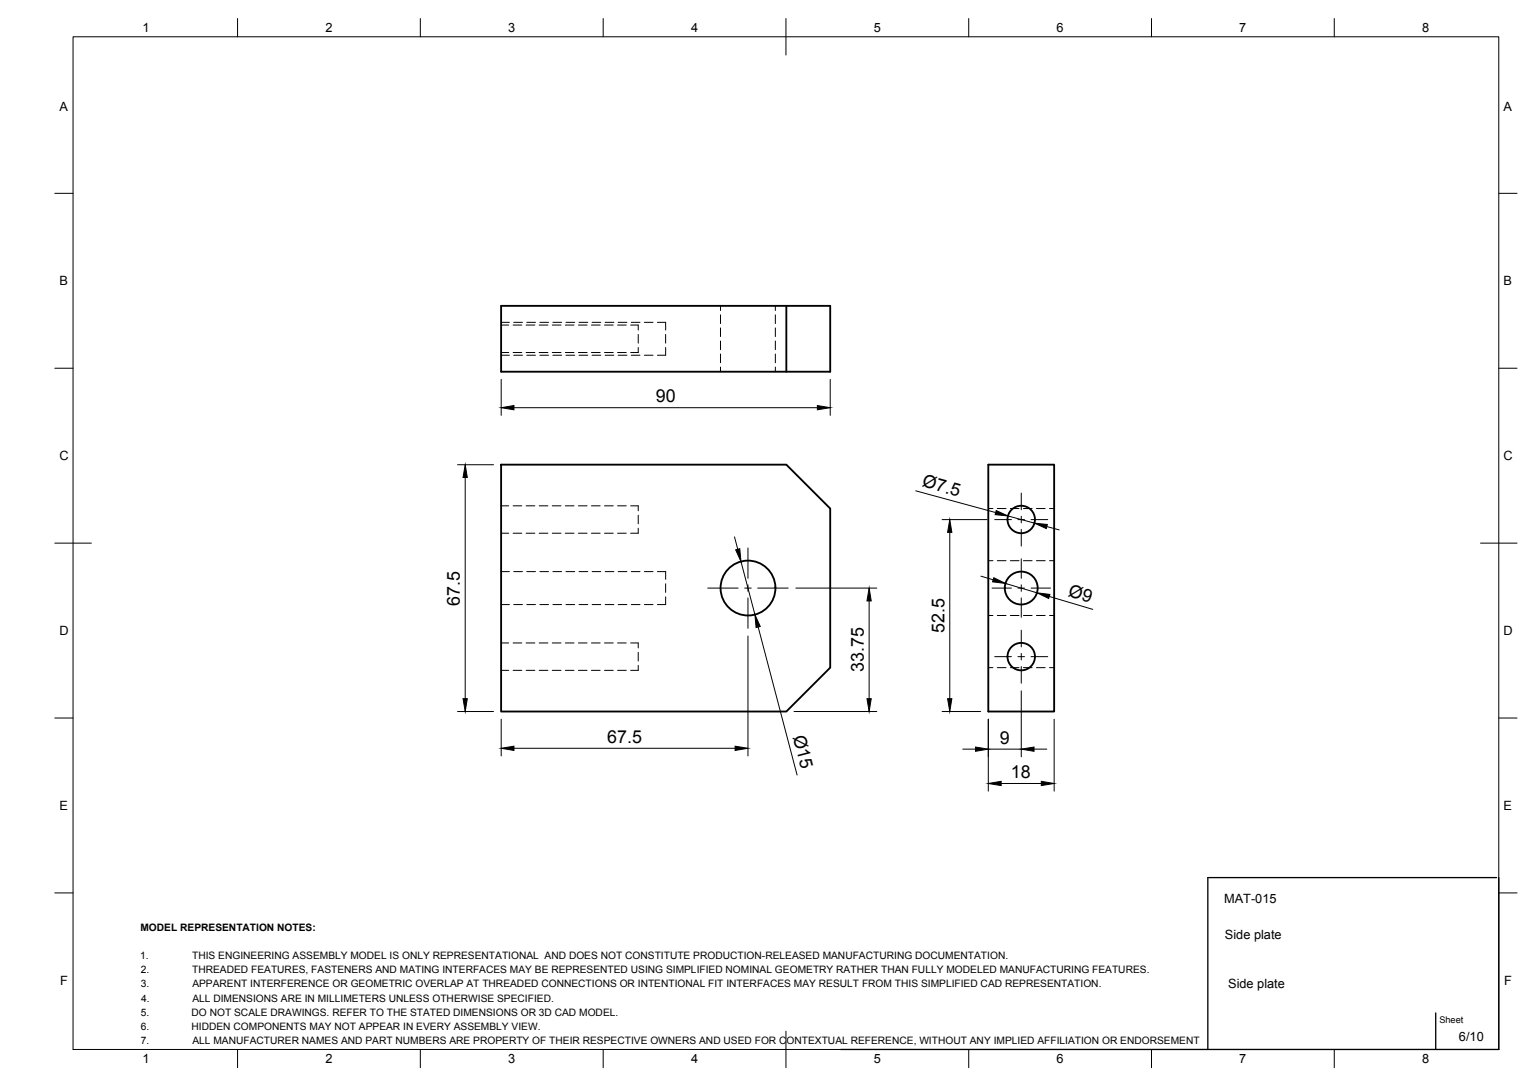
ISO-10303-21;
HEADER;
/* Generated by software containing ST-Developer
 * from STEP Tools, Inc. (www.steptools.com) 
 */

FILE_DESCRIPTION(
/* description */ ('STEP AP214'),
/* implementation_level */ '2;1');

FILE_NAME(
/* name */ 'Side Plate.step',
/* time_stamp */ '2026-11-14T06:03:18-08:00',
/* author */ (''),
/* organization */ (''),
/* preprocessor_version */ 'ST-DEVELOPER v20.2',
/* originating_system */ 'Autodesk Translation Framework v15.17.0.0',
/* authorisation */ '');

FILE_SCHEMA (('AUTOMOTIVE_DESIGN { 1 0 10303 214 3 1 1 }'));
ENDSEC;

DATA;
#10=MECHANICAL_DESIGN_GEOMETRIC_PRESENTATION_REPRESENTATION('',(#74),#3206);
#58=SHAPE_REPRESENTATION_RELATIONSHIP('SRR','None',#3241,#66);
#66=ADVANCED_BREP_SHAPE_REPRESENTATION('',(#82),#3200);
#74=STYLED_ITEM('',(#3288),#82);
#82=MANIFOLD_SOLID_BREP('Body1',#1781);
#98=PLANE('',#1938);
#99=PLANE('',#1939);
#100=PLANE('',#1940);
#101=PLANE('',#1941);
#102=PLANE('',#1942);
#103=PLANE('',#1943);
#104=PLANE('',#1944);
#105=PLANE('',#1945);
#106=PLANE('',#1946);
#107=PLANE('',#1947);
#108=PLANE('',#1948);
#155=FACE_BOUND('',#647,.T.);
#156=FACE_BOUND('',#649,.T.);
#157=FACE_BOUND('',#652,.T.);
#158=FACE_BOUND('',#653,.T.);
#159=FACE_BOUND('',#654,.T.);
#202=LINE('',#2786,#347);
#203=LINE('',#2792,#348);
#204=LINE('',#2798,#349);
#205=LINE('',#2804,#350);
#206=LINE('',#2809,#351);
#207=LINE('',#2811,#352);
#208=LINE('',#2813,#353);
#209=LINE('',#2815,#354);
#210=LINE('',#2817,#355);
#211=LINE('',#2818,#356);
#212=LINE('',#2822,#357);
#213=LINE('',#2824,#358);
#214=LINE('',#2826,#359);
#215=LINE('',#2828,#360);
#216=LINE('',#2830,#361);
#217=LINE('',#2831,#362);
#218=LINE('',#2833,#363);
#219=LINE('',#2834,#364);
#220=LINE('',#2836,#365);
#221=LINE('',#2838,#366);
#222=LINE('',#2840,#367);
#223=LINE('',#2841,#368);
#347=VECTOR('',#2193,4.5);
#348=VECTOR('',#2200,3.75);
#349=VECTOR('',#2207,3.75);
#350=VECTOR('',#2214,7.50000000000001);
#351=VECTOR('',#2219,1000.);
#352=VECTOR('',#2220,1000.);
#353=VECTOR('',#2221,1000.);
#354=VECTOR('',#2222,1000.);
#355=VECTOR('',#2223,1000.);
#356=VECTOR('',#2224,1000.);
#357=VECTOR('',#2227,1000.);
#358=VECTOR('',#2228,1000.);
#359=VECTOR('',#2229,1000.);
#360=VECTOR('',#2230,1000.);
#361=VECTOR('',#2231,1000.);
#362=VECTOR('',#2232,1000.);
#363=VECTOR('',#2235,1000.);
#364=VECTOR('',#2236,1000.);
#365=VECTOR('',#2239,1000.);
#366=VECTOR('',#2242,1000.);
#367=VECTOR('',#2245,1000.);
#368=VECTOR('',#2246,1000.);
#485=CYLINDRICAL_SURFACE('',#1926,4.5);
#486=CYLINDRICAL_SURFACE('',#1929,3.75);
#487=CYLINDRICAL_SURFACE('',#1932,3.75);
#488=CYLINDRICAL_SURFACE('',#1935,7.50000000000001);
#534=FACE_OUTER_BOUND('',#642,.T.);
#535=FACE_OUTER_BOUND('',#643,.T.);
#536=FACE_OUTER_BOUND('',#644,.T.);
#537=FACE_OUTER_BOUND('',#645,.T.);
#538=FACE_OUTER_BOUND('',#646,.T.);
#539=FACE_OUTER_BOUND('',#648,.T.);
#540=FACE_OUTER_BOUND('',#650,.T.);
#541=FACE_OUTER_BOUND('',#651,.T.);
#542=FACE_OUTER_BOUND('',#655,.T.);
#543=FACE_OUTER_BOUND('',#656,.T.);
#544=FACE_OUTER_BOUND('',#657,.T.);
#545=FACE_OUTER_BOUND('',#658,.T.);
#546=FACE_OUTER_BOUND('',#659,.T.);
#547=FACE_OUTER_BOUND('',#660,.T.);
#548=FACE_OUTER_BOUND('',#661,.T.);
#642=EDGE_LOOP('',(#1301,#1302,#1303,#1304));
#643=EDGE_LOOP('',(#1305,#1306,#1307,#1308));
#644=EDGE_LOOP('',(#1309,#1310,#1311,#1312));
#645=EDGE_LOOP('',(#1313,#1314,#1315,#1316));
#646=EDGE_LOOP('',(#1317,#1318,#1319,#1320,#1321,#1322));
#647=EDGE_LOOP('',(#1323));
#648=EDGE_LOOP('',(#1324,#1325,#1326,#1327,#1328,#1329));
#649=EDGE_LOOP('',(#1330));
#650=EDGE_LOOP('',(#1331,#1332,#1333,#1334));
#651=EDGE_LOOP('',(#1335,#1336,#1337,#1338));
#652=EDGE_LOOP('',(#1339));
#653=EDGE_LOOP('',(#1340));
#654=EDGE_LOOP('',(#1341));
#655=EDGE_LOOP('',(#1342,#1343,#1344,#1345));
#656=EDGE_LOOP('',(#1346,#1347,#1348,#1349));
#657=EDGE_LOOP('',(#1350,#1351,#1352,#1353));
#658=EDGE_LOOP('',(#1354,#1355,#1356,#1357));
#659=EDGE_LOOP('',(#1358));
#660=EDGE_LOOP('',(#1359));
#661=EDGE_LOOP('',(#1360));
#777=CIRCLE('',#1927,4.5);
#778=CIRCLE('',#1928,4.5);
#779=CIRCLE('',#1930,3.75);
#780=CIRCLE('',#1931,3.75);
#781=CIRCLE('',#1933,3.75);
#782=CIRCLE('',#1934,3.75);
#783=CIRCLE('',#1936,7.50000000000001);
#784=CIRCLE('',#1937,7.50000000000001);
#862=VERTEX_POINT('',#2783);
#863=VERTEX_POINT('',#2785);
#864=VERTEX_POINT('',#2789);
#865=VERTEX_POINT('',#2791);
#866=VERTEX_POINT('',#2795);
#867=VERTEX_POINT('',#2797);
#868=VERTEX_POINT('',#2801);
#869=VERTEX_POINT('',#2803);
#870=VERTEX_POINT('',#2807);
#871=VERTEX_POINT('',#2808);
#872=VERTEX_POINT('',#2810);
#873=VERTEX_POINT('',#2812);
#874=VERTEX_POINT('',#2814);
#875=VERTEX_POINT('',#2816);
#876=VERTEX_POINT('',#2820);
#877=VERTEX_POINT('',#2821);
#878=VERTEX_POINT('',#2823);
#879=VERTEX_POINT('',#2825);
#880=VERTEX_POINT('',#2827);
#881=VERTEX_POINT('',#2829);
#1029=EDGE_CURVE('',#862,#862,#777,.T.);
#1030=EDGE_CURVE('',#862,#863,#202,.T.);
#1031=EDGE_CURVE('',#863,#863,#778,.T.);
#1032=EDGE_CURVE('',#864,#864,#779,.T.);
#1033=EDGE_CURVE('',#864,#865,#203,.T.);
#1034=EDGE_CURVE('',#865,#865,#780,.T.);
#1035=EDGE_CURVE('',#866,#866,#781,.T.);
#1036=EDGE_CURVE('',#866,#867,#204,.T.);
#1037=EDGE_CURVE('',#867,#867,#782,.T.);
#1038=EDGE_CURVE('',#868,#868,#783,.T.);
#1039=EDGE_CURVE('',#868,#869,#205,.T.);
#1040=EDGE_CURVE('',#869,#869,#784,.T.);
#1041=EDGE_CURVE('',#870,#871,#206,.T.);
#1042=EDGE_CURVE('',#871,#872,#207,.T.);
#1043=EDGE_CURVE('',#872,#873,#208,.T.);
#1044=EDGE_CURVE('',#873,#874,#209,.T.);
#1045=EDGE_CURVE('',#874,#875,#210,.T.);
#1046=EDGE_CURVE('',#875,#870,#211,.T.);
#1047=EDGE_CURVE('',#876,#877,#212,.T.);
#1048=EDGE_CURVE('',#876,#878,#213,.T.);
#1049=EDGE_CURVE('',#879,#878,#214,.T.);
#1050=EDGE_CURVE('',#879,#880,#215,.T.);
#1051=EDGE_CURVE('',#881,#880,#216,.T.);
#1052=EDGE_CURVE('',#877,#881,#217,.T.);
#1053=EDGE_CURVE('',#872,#876,#218,.T.);
#1054=EDGE_CURVE('',#873,#877,#219,.T.);
#1055=EDGE_CURVE('',#874,#881,#220,.T.);
#1056=EDGE_CURVE('',#880,#875,#221,.T.);
#1057=EDGE_CURVE('',#878,#871,#222,.T.);
#1058=EDGE_CURVE('',#870,#879,#223,.T.);
#1301=ORIENTED_EDGE('',*,*,#1029,.F.);
#1302=ORIENTED_EDGE('',*,*,#1030,.T.);
#1303=ORIENTED_EDGE('',*,*,#1031,.T.);
#1304=ORIENTED_EDGE('',*,*,#1030,.F.);
#1305=ORIENTED_EDGE('',*,*,#1032,.F.);
#1306=ORIENTED_EDGE('',*,*,#1033,.T.);
#1307=ORIENTED_EDGE('',*,*,#1034,.T.);
#1308=ORIENTED_EDGE('',*,*,#1033,.F.);
#1309=ORIENTED_EDGE('',*,*,#1035,.F.);
#1310=ORIENTED_EDGE('',*,*,#1036,.T.);
#1311=ORIENTED_EDGE('',*,*,#1037,.T.);
#1312=ORIENTED_EDGE('',*,*,#1036,.F.);
#1313=ORIENTED_EDGE('',*,*,#1038,.T.);
#1314=ORIENTED_EDGE('',*,*,#1039,.T.);
#1315=ORIENTED_EDGE('',*,*,#1040,.F.);
#1316=ORIENTED_EDGE('',*,*,#1039,.F.);
#1317=ORIENTED_EDGE('',*,*,#1041,.T.);
#1318=ORIENTED_EDGE('',*,*,#1042,.T.);
#1319=ORIENTED_EDGE('',*,*,#1043,.T.);
#1320=ORIENTED_EDGE('',*,*,#1044,.T.);
#1321=ORIENTED_EDGE('',*,*,#1045,.T.);
#1322=ORIENTED_EDGE('',*,*,#1046,.T.);
#1323=ORIENTED_EDGE('',*,*,#1038,.F.);
#1324=ORIENTED_EDGE('',*,*,#1047,.F.);
#1325=ORIENTED_EDGE('',*,*,#1048,.T.);
#1326=ORIENTED_EDGE('',*,*,#1049,.F.);
#1327=ORIENTED_EDGE('',*,*,#1050,.T.);
#1328=ORIENTED_EDGE('',*,*,#1051,.F.);
#1329=ORIENTED_EDGE('',*,*,#1052,.F.);
#1330=ORIENTED_EDGE('',*,*,#1040,.T.);
#1331=ORIENTED_EDGE('',*,*,#1043,.F.);
#1332=ORIENTED_EDGE('',*,*,#1053,.T.);
#1333=ORIENTED_EDGE('',*,*,#1047,.T.);
#1334=ORIENTED_EDGE('',*,*,#1054,.F.);
#1335=ORIENTED_EDGE('',*,*,#1052,.T.);
#1336=ORIENTED_EDGE('',*,*,#1055,.F.);
#1337=ORIENTED_EDGE('',*,*,#1044,.F.);
#1338=ORIENTED_EDGE('',*,*,#1054,.T.);
#1339=ORIENTED_EDGE('',*,*,#1031,.F.);
#1340=ORIENTED_EDGE('',*,*,#1034,.F.);
#1341=ORIENTED_EDGE('',*,*,#1037,.F.);
#1342=ORIENTED_EDGE('',*,*,#1051,.T.);
#1343=ORIENTED_EDGE('',*,*,#1056,.T.);
#1344=ORIENTED_EDGE('',*,*,#1045,.F.);
#1345=ORIENTED_EDGE('',*,*,#1055,.T.);
#1346=ORIENTED_EDGE('',*,*,#1049,.T.);
#1347=ORIENTED_EDGE('',*,*,#1057,.T.);
#1348=ORIENTED_EDGE('',*,*,#1041,.F.);
#1349=ORIENTED_EDGE('',*,*,#1058,.T.);
#1350=ORIENTED_EDGE('',*,*,#1042,.F.);
#1351=ORIENTED_EDGE('',*,*,#1057,.F.);
#1352=ORIENTED_EDGE('',*,*,#1048,.F.);
#1353=ORIENTED_EDGE('',*,*,#1053,.F.);
#1354=ORIENTED_EDGE('',*,*,#1046,.F.);
#1355=ORIENTED_EDGE('',*,*,#1056,.F.);
#1356=ORIENTED_EDGE('',*,*,#1050,.F.);
#1357=ORIENTED_EDGE('',*,*,#1058,.F.);
#1358=ORIENTED_EDGE('',*,*,#1035,.T.);
#1359=ORIENTED_EDGE('',*,*,#1032,.T.);
#1360=ORIENTED_EDGE('',*,*,#1029,.T.);
#1701=ADVANCED_FACE('',(#534),#485,.F.);
#1702=ADVANCED_FACE('',(#535),#486,.F.);
#1703=ADVANCED_FACE('',(#536),#487,.F.);
#1704=ADVANCED_FACE('',(#537),#488,.F.);
#1705=ADVANCED_FACE('',(#538,#155),#98,.T.);
#1706=ADVANCED_FACE('',(#539,#156),#99,.F.);
#1707=ADVANCED_FACE('',(#540),#100,.F.);
#1708=ADVANCED_FACE('',(#541,#157,#158,#159),#101,.F.);
#1709=ADVANCED_FACE('',(#542),#102,.F.);
#1710=ADVANCED_FACE('',(#543),#103,.F.);
#1711=ADVANCED_FACE('',(#544),#104,.F.);
#1712=ADVANCED_FACE('',(#545),#105,.F.);
#1713=ADVANCED_FACE('',(#546),#106,.T.);
#1714=ADVANCED_FACE('',(#547),#107,.T.);
#1715=ADVANCED_FACE('',(#548),#108,.T.);
#1781=CLOSED_SHELL('',(#1701,#1702,#1703,#1704,#1705,#1706,#1707,#1708,
#1709,#1710,#1711,#1712,#1713,#1714,#1715));
#1925=AXIS2_PLACEMENT_3D('',#2781,#2187,#2188);
#1926=AXIS2_PLACEMENT_3D('',#2782,#2189,#2190);
#1927=AXIS2_PLACEMENT_3D('',#2784,#2191,#2192);
#1928=AXIS2_PLACEMENT_3D('',#2787,#2194,#2195);
#1929=AXIS2_PLACEMENT_3D('',#2788,#2196,#2197);
#1930=AXIS2_PLACEMENT_3D('',#2790,#2198,#2199);
#1931=AXIS2_PLACEMENT_3D('',#2793,#2201,#2202);
#1932=AXIS2_PLACEMENT_3D('',#2794,#2203,#2204);
#1933=AXIS2_PLACEMENT_3D('',#2796,#2205,#2206);
#1934=AXIS2_PLACEMENT_3D('',#2799,#2208,#2209);
#1935=AXIS2_PLACEMENT_3D('',#2800,#2210,#2211);
#1936=AXIS2_PLACEMENT_3D('',#2802,#2212,#2213);
#1937=AXIS2_PLACEMENT_3D('',#2805,#2215,#2216);
#1938=AXIS2_PLACEMENT_3D('',#2806,#2217,#2218);
#1939=AXIS2_PLACEMENT_3D('',#2819,#2225,#2226);
#1940=AXIS2_PLACEMENT_3D('',#2832,#2233,#2234);
#1941=AXIS2_PLACEMENT_3D('',#2835,#2237,#2238);
#1942=AXIS2_PLACEMENT_3D('',#2837,#2240,#2241);
#1943=AXIS2_PLACEMENT_3D('',#2839,#2243,#2244);
#1944=AXIS2_PLACEMENT_3D('',#2842,#2247,#2248);
#1945=AXIS2_PLACEMENT_3D('',#2843,#2249,#2250);
#1946=AXIS2_PLACEMENT_3D('',#2844,#2251,#2252);
#1947=AXIS2_PLACEMENT_3D('',#2845,#2253,#2254);
#1948=AXIS2_PLACEMENT_3D('',#2846,#2255,#2256);
#2187=DIRECTION('axis',(0.,0.,1.));
#2188=DIRECTION('refdir',(1.,0.,0.));
#2189=DIRECTION('center_axis',(1.04083408558608E-17,-1.,-1.5392995080515E-31));
#2190=DIRECTION('ref_axis',(-1.60215539590589E-48,1.5392995080515E-31,-1.));
#2191=DIRECTION('center_axis',(1.04083408558608E-17,-1.,-1.5392995080515E-31));
#2192=DIRECTION('ref_axis',(-1.60215539590589E-48,1.5392995080515E-31,-1.));
#2193=DIRECTION('',(1.04083408558608E-17,-1.,-1.5392995080515E-31));
#2194=DIRECTION('center_axis',(1.04083408558608E-17,-1.,-1.5392995080515E-31));
#2195=DIRECTION('ref_axis',(-1.60215539590589E-48,1.5392995080515E-31,-1.));
#2196=DIRECTION('center_axis',(1.04083408558608E-17,-1.,-1.5392995080515E-31));
#2197=DIRECTION('ref_axis',(-1.60215539590589E-48,1.5392995080515E-31,-1.));
#2198=DIRECTION('center_axis',(1.04083408558608E-17,-1.,-1.5392995080515E-31));
#2199=DIRECTION('ref_axis',(-1.60215539590589E-48,1.5392995080515E-31,-1.));
#2200=DIRECTION('',(1.04083408558608E-17,-1.,-1.5392995080515E-31));
#2201=DIRECTION('center_axis',(1.04083408558608E-17,-1.,-1.5392995080515E-31));
#2202=DIRECTION('ref_axis',(-1.60215539590589E-48,1.5392995080515E-31,-1.));
#2203=DIRECTION('center_axis',(1.04083408558608E-17,-1.,-1.5392995080515E-31));
#2204=DIRECTION('ref_axis',(-1.60215539590589E-48,1.5392995080515E-31,-1.));
#2205=DIRECTION('center_axis',(1.04083408558608E-17,-1.,-1.5392995080515E-31));
#2206=DIRECTION('ref_axis',(-1.60215539590589E-48,1.5392995080515E-31,-1.));
#2207=DIRECTION('',(1.04083408558608E-17,-1.,-1.5392995080515E-31));
#2208=DIRECTION('center_axis',(1.04083408558608E-17,-1.,-1.5392995080515E-31));
#2209=DIRECTION('ref_axis',(-1.60215539590589E-48,1.5392995080515E-31,-1.));
#2210=DIRECTION('center_axis',(6.16297582203915E-33,-1.47526233740062E-31,
-1.));
#2211=DIRECTION('ref_axis',(-1.,-9.09200611656501E-64,-6.16297582203915E-33));
#2212=DIRECTION('center_axis',(-6.16297582203915E-33,1.47526233740062E-31,
1.));
#2213=DIRECTION('ref_axis',(1.,9.09200611656501E-64,6.16297582203915E-33));
#2214=DIRECTION('',(6.16297582203915E-33,-1.47526233740062E-31,-1.));
#2215=DIRECTION('center_axis',(-6.16297582203915E-33,1.47526233740062E-31,
1.));
#2216=DIRECTION('ref_axis',(1.,9.09200611656501E-64,6.16297582203915E-33));
#2217=DIRECTION('center_axis',(4.62223186652936E-33,1.47526233740062E-31,
1.));
#2218=DIRECTION('ref_axis',(1.,1.04083408558608E-17,-4.62223186652936E-33));
#2219=DIRECTION('',(-1.,-1.04083408558608E-17,6.16297582203915E-33));
#2220=DIRECTION('',(-0.707106781186549,-0.707106781186546,-7.08742219534503E-32));
#2221=DIRECTION('',(1.04083408558608E-17,-1.,-1.5392995080515E-31));
#2222=DIRECTION('',(1.,1.04083408558608E-17,-6.16297582203915E-33));
#2223=DIRECTION('',(-1.04083408558608E-17,1.,1.5383365430793E-31));
#2224=DIRECTION('',(-0.707106781186546,0.707106781186549,7.70371977754894E-32));
#2225=DIRECTION('center_axis',(4.62223186652936E-33,1.47526233740062E-31,
1.));
#2226=DIRECTION('ref_axis',(1.,1.04083408558608E-17,-4.62223186652936E-33));
#2227=DIRECTION('',(1.04083408558608E-17,-1.,-1.5392995080515E-31));
#2228=DIRECTION('',(0.707106781186549,0.707106781186546,7.08742219534503E-32));
#2229=DIRECTION('',(-1.,-1.04083408558608E-17,6.16297582203915E-33));
#2230=DIRECTION('',(0.707106781186546,-0.707106781186549,-7.70371977754894E-32));
#2231=DIRECTION('',(-1.04083408558608E-17,1.,1.5392995080515E-31));
#2232=DIRECTION('',(1.,1.04083408558608E-17,-6.16297582203915E-33));
#2233=DIRECTION('center_axis',(1.,1.04083408558608E-17,6.16297582203915E-33));
#2234=DIRECTION('ref_axis',(6.16297582203915E-33,-1.47526233740062E-31,
-1.));
#2235=DIRECTION('',(6.16297582203915E-33,-1.47526233740062E-31,-1.));
#2236=DIRECTION('',(6.16297582203915E-33,-1.47526233740062E-31,-1.));
#2237=DIRECTION('center_axis',(-1.04083408558608E-17,1.,-1.47526233740062E-31));
#2238=DIRECTION('ref_axis',(-6.16297582203915E-33,1.47526233740062E-31,
1.));
#2239=DIRECTION('',(6.16297582203915E-33,-1.47526233740062E-31,-1.));
#2240=DIRECTION('center_axis',(-1.,-1.04083408558608E-17,-6.16297582203915E-33));
#2241=DIRECTION('ref_axis',(-6.16297582203915E-33,1.47526233740062E-31,
1.));
#2242=DIRECTION('',(-6.16297582203915E-33,1.47526233740062E-31,1.));
#2243=DIRECTION('center_axis',(1.04083408558608E-17,-1.,1.47526233740062E-31));
#2244=DIRECTION('ref_axis',(6.16297582203915E-33,-1.47526233740062E-31,
-1.));
#2245=DIRECTION('',(-6.16297582203915E-33,1.47526233740062E-31,1.));
#2246=DIRECTION('',(6.16297582203915E-33,-1.47526233740062E-31,-1.));
#2247=DIRECTION('center_axis',(0.707106781186546,-0.707106781186549,1.08674682276562E-31));
#2248=DIRECTION('ref_axis',(6.16297582203915E-33,-1.47526233740062E-31,
-1.));
#2249=DIRECTION('center_axis',(-0.707106781186549,-0.707106781186546,9.99589182844569E-32));
#2250=DIRECTION('ref_axis',(6.16297582203915E-33,-1.47526233740062E-31,
-1.));
#2251=DIRECTION('center_axis',(1.04083408558608E-17,-1.,1.47526233740062E-31));
#2252=DIRECTION('ref_axis',(6.16297582203915E-33,-1.47526233740062E-31,
-1.));
#2253=DIRECTION('center_axis',(1.04083408558608E-17,-1.,1.47526233740062E-31));
#2254=DIRECTION('ref_axis',(6.16297582203915E-33,-1.47526233740062E-31,
-1.));
#2255=DIRECTION('center_axis',(1.04083408558608E-17,-1.,1.47526233740062E-31));
#2256=DIRECTION('ref_axis',(6.16297582203915E-33,-1.47526233740062E-31,
-1.));
#2781=CARTESIAN_POINT('',(0.,0.,0.));
#2782=CARTESIAN_POINT('Origin',(22.5,30.0905269290172,6.));
#2783=CARTESIAN_POINT('',(22.5,30.0905269290172,10.5));
#2784=CARTESIAN_POINT('Origin',(22.5,30.0905269290172,6.));
#2785=CARTESIAN_POINT('',(22.5,-14.9094730709829,10.5));
#2786=CARTESIAN_POINT('',(22.5,30.0905269290172,10.5));
#2787=CARTESIAN_POINT('Origin',(22.5,-14.9094730709829,6.));
#2788=CARTESIAN_POINT('Origin',(41.25,22.5905269290171,6.));
#2789=CARTESIAN_POINT('',(41.25,22.5905269290171,9.75000000000001));
#2790=CARTESIAN_POINT('Origin',(41.25,22.5905269290171,6.));
#2791=CARTESIAN_POINT('',(41.25,-14.9094730709829,9.75000000000001));
#2792=CARTESIAN_POINT('',(41.25,22.5905269290171,9.75000000000001));
#2793=CARTESIAN_POINT('Origin',(41.25,-14.9094730709829,6.));
#2794=CARTESIAN_POINT('Origin',(3.74999999999999,22.5905269290171,6.));
#2795=CARTESIAN_POINT('',(3.74999999999999,22.5905269290171,9.75));
#2796=CARTESIAN_POINT('Origin',(3.74999999999999,22.5905269290171,6.));
#2797=CARTESIAN_POINT('',(3.74999999999999,-14.9094730709828,9.75));
#2798=CARTESIAN_POINT('',(3.74999999999999,22.5905269290171,9.75));
#2799=CARTESIAN_POINT('Origin',(3.74999999999992,-14.9094730709828,6.));
#2800=CARTESIAN_POINT('Origin',(22.5,52.5905269290171,15.));
#2801=CARTESIAN_POINT('',(30.,52.5905269290171,15.));
#2802=CARTESIAN_POINT('Origin',(22.5,52.5905269290171,15.));
#2803=CARTESIAN_POINT('',(30.,52.5905269290171,-3.));
#2804=CARTESIAN_POINT('',(30.,52.5905269290171,15.));
#2805=CARTESIAN_POINT('Origin',(22.5,52.5905269290171,-3.));
#2806=CARTESIAN_POINT('Origin',(-11.2500000000001,-14.9094730709829,15.));
#2807=CARTESIAN_POINT('',(44.25,75.0905269290171,15.));
#2808=CARTESIAN_POINT('',(0.750000000000084,75.0905269290172,15.));
#2809=CARTESIAN_POINT('',(56.25,75.0905269290171,15.));
#2810=CARTESIAN_POINT('',(-11.25,63.0905269290172,15.));
#2811=CARTESIAN_POINT('',(-50.2500000000001,24.0905269290173,15.));
#2812=CARTESIAN_POINT('',(-11.2500000000001,-14.9094730709829,15.));
#2813=CARTESIAN_POINT('',(-11.2500000000001,75.0905269290171,15.));
#2814=CARTESIAN_POINT('',(56.25,-14.9094730709829,15.));
#2815=CARTESIAN_POINT('',(-11.2500000000001,-14.9094730709829,15.));
#2816=CARTESIAN_POINT('',(56.25,63.0905269290171,15.));
#2817=CARTESIAN_POINT('',(56.25,-14.9094730709829,15.));
#2818=CARTESIAN_POINT('',(61.5000000000001,57.840526929017,15.));
#2819=CARTESIAN_POINT('Origin',(-11.2500000000001,-14.9094730709829,-3.));
#2820=CARTESIAN_POINT('',(-11.25,63.0905269290171,-3.));
#2821=CARTESIAN_POINT('',(-11.2500000000001,-14.9094730709829,-3.));
#2822=CARTESIAN_POINT('',(-11.2500000000001,75.0905269290171,-3.));
#2823=CARTESIAN_POINT('',(0.75000000000007,75.0905269290171,-3.));
#2824=CARTESIAN_POINT('',(-11.25,63.0905269290171,-3.));
#2825=CARTESIAN_POINT('',(44.25,75.0905269290171,-3.));
#2826=CARTESIAN_POINT('',(56.25,75.0905269290171,-3.));
#2827=CARTESIAN_POINT('',(56.25,63.0905269290171,-3.));
#2828=CARTESIAN_POINT('',(44.25,75.0905269290171,-3.));
#2829=CARTESIAN_POINT('',(56.25,-14.9094730709829,-3.));
#2830=CARTESIAN_POINT('',(56.25,52.5905269290171,-3.));
#2831=CARTESIAN_POINT('',(-11.2500000000001,-14.9094730709829,-3.));
#2832=CARTESIAN_POINT('Origin',(-11.2500000000001,75.0905269290171,15.));
#2833=CARTESIAN_POINT('',(-11.25,63.0905269290171,15.));
#2834=CARTESIAN_POINT('',(-11.2500000000001,-14.9094730709829,15.));
#2835=CARTESIAN_POINT('Origin',(-11.2500000000001,-14.9094730709829,15.));
#2836=CARTESIAN_POINT('',(56.25,-14.9094730709829,15.));
#2837=CARTESIAN_POINT('Origin',(56.25,52.5905269290171,15.));
#2838=CARTESIAN_POINT('',(56.25,63.0905269290171,15.));
#2839=CARTESIAN_POINT('Origin',(56.25,75.0905269290171,15.));
#2840=CARTESIAN_POINT('',(0.750000000000056,75.0905269290171,15.));
#2841=CARTESIAN_POINT('',(44.25,75.0905269290171,15.));
#2842=CARTESIAN_POINT('Origin',(-11.25,63.0905269290171,15.));
#2843=CARTESIAN_POINT('Origin',(44.25,75.0905269290171,15.));
#2844=CARTESIAN_POINT('Origin',(3.74999999999999,22.5905269290171,6.));
#2845=CARTESIAN_POINT('Origin',(41.25,22.5905269290171,6.));
#2846=CARTESIAN_POINT('Origin',(22.5,30.0905269290172,6.));
#3190=UNCERTAINTY_MEASURE_WITH_UNIT(LENGTH_MEASURE(0.01),#3207,
'DISTANCE_ACCURACY_VALUE',
'Maximum model space distance between geometric entities at asserted c
onnectivities');
#3196=UNCERTAINTY_MEASURE_WITH_UNIT(LENGTH_MEASURE(0.01),#3207,
'DISTANCE_ACCURACY_VALUE',
'Maximum model space distance between geometric entities at asserted c
onnectivities');
#3200=(
GEOMETRIC_REPRESENTATION_CONTEXT(3)
GLOBAL_UNCERTAINTY_ASSIGNED_CONTEXT((#3190))
GLOBAL_UNIT_ASSIGNED_CONTEXT((#3207,#3209,#3210))
REPRESENTATION_CONTEXT('','3D')
);
#3206=(
GEOMETRIC_REPRESENTATION_CONTEXT(3)
GLOBAL_UNCERTAINTY_ASSIGNED_CONTEXT((#3196))
GLOBAL_UNIT_ASSIGNED_CONTEXT((#3207,#3209,#3210))
REPRESENTATION_CONTEXT('','3D')
);
#3207=(
LENGTH_UNIT()
NAMED_UNIT(*)
SI_UNIT(.MILLI.,.METRE.)
);
#3209=(
NAMED_UNIT(*)
PLANE_ANGLE_UNIT()
SI_UNIT($,.RADIAN.)
);
#3210=(
NAMED_UNIT(*)
SI_UNIT($,.STERADIAN.)
SOLID_ANGLE_UNIT()
);
#3214=SHAPE_DEFINITION_REPRESENTATION(#3223,#3241);
#3223=PRODUCT_DEFINITION_SHAPE('',$,#3251);
#3241=SHAPE_REPRESENTATION('',(#1925),#3200);
#3247=PRODUCT_DEFINITION_CONTEXT('part definition',#3276,'design');
#3251=PRODUCT_DEFINITION('Side plate','Side Plate',#3260,#3247);
#3260=PRODUCT_DEFINITION_FORMATION('',$,#3281);
#3276=APPLICATION_CONTEXT(
'Core Data for Automotive Mechanical Design Process');
#3277=PRODUCT_CONTEXT('part definition',#3276,'mechanical');
#3281=PRODUCT('Side plate','Side Plate','Side plate',(#3277));
#3288=PRESENTATION_STYLE_ASSIGNMENT((#3292));
#3292=SURFACE_STYLE_USAGE(.BOTH.,#3296);
#3296=SURFACE_SIDE_STYLE('',(#3300));
#3300=SURFACE_STYLE_FILL_AREA(#3304);
#3304=FILL_AREA_STYLE('Opaque(61,176,222)',(#3308));
#3308=FILL_AREA_STYLE_COLOUR('Opaque(61,176,222)',#3312);
#3312=COLOUR_RGB('Opaque(61,176,222)',0.23921568627451,0.690196078431373,
0.870588235294118);
ENDSEC;
END-ISO-10303-21;
